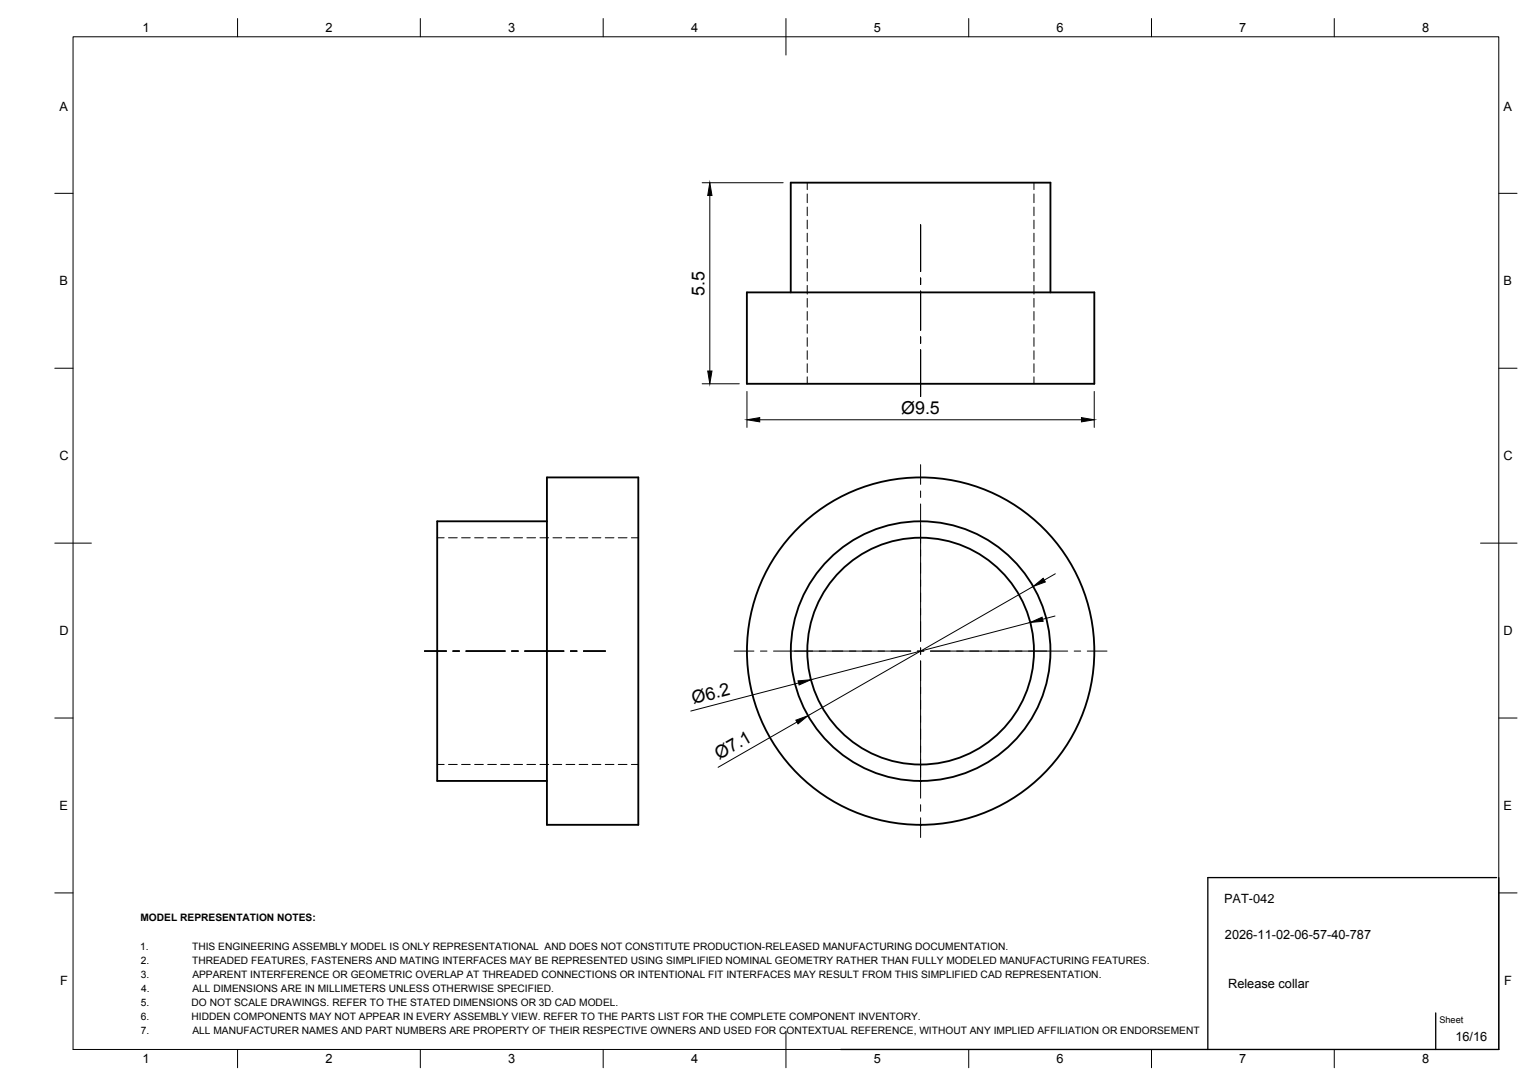
ISO-10303-21;
HEADER;
/* Generated by software containing ST-Developer
 * from STEP Tools, Inc. (www.steptools.com) 
 */

FILE_DESCRIPTION(
/* description */ ('Manifold and mounting hardware'),
/* implementation_level */ '2;1');

FILE_NAME(
/* name */ 'Release collar.step',
/* time_stamp */ '2026-10-28T21:46:49-07:00',
/* author */ (''),
/* organization */ (''),
/* preprocessor_version */ 'ST-DEVELOPER v20.2',
/* originating_system */ 'Autodesk Translation Framework v15.17.0.0',
/* authorisation */ '');

FILE_SCHEMA (('AUTOMOTIVE_DESIGN { 1 0 10303 214 3 1 1 }'));
ENDSEC;

DATA;
#10=MECHANICAL_DESIGN_GEOMETRIC_PRESENTATION_REPRESENTATION('',(#160),#5638);
#132=SHAPE_REPRESENTATION_RELATIONSHIP('SRR','None',#5712,#146);
#146=ADVANCED_BREP_SHAPE_REPRESENTATION('',(#174),#5634);
#160=STYLED_ITEM('',(#5874),#174);
#174=MANIFOLD_SOLID_BREP('Body1',#3150);
#247=FACE_BOUND('',#746,.T.);
#248=FACE_BOUND('',#749,.T.);
#249=FACE_BOUND('',#752,.T.);
#323=CYLINDRICAL_SURFACE('',#3604,0.475);
#324=CYLINDRICAL_SURFACE('',#3608,0.355);
#325=CYLINDRICAL_SURFACE('',#3612,0.31);
#490=FACE_OUTER_BOUND('',#745,.T.);
#491=FACE_OUTER_BOUND('',#747,.T.);
#492=FACE_OUTER_BOUND('',#748,.T.);
#493=FACE_OUTER_BOUND('',#750,.T.);
#494=FACE_OUTER_BOUND('',#751,.T.);
#495=FACE_OUTER_BOUND('',#753,.T.);
#745=EDGE_LOOP('',(#2740));
#746=EDGE_LOOP('',(#2741));
#747=EDGE_LOOP('',(#2742,#2743,#2744,#2745));
#748=EDGE_LOOP('',(#2746));
#749=EDGE_LOOP('',(#2747));
#750=EDGE_LOOP('',(#2748,#2749,#2750,#2751));
#751=EDGE_LOOP('',(#2752));
#752=EDGE_LOOP('',(#2753));
#753=EDGE_LOOP('',(#2754,#2755,#2756,#2757));
#880=CIRCLE('',#3602,0.475);
#881=CIRCLE('',#3603,0.31);
#882=CIRCLE('',#3605,0.475);
#883=CIRCLE('',#3607,0.355);
#884=CIRCLE('',#3609,0.355);
#885=CIRCLE('',#3611,0.31);
#1122=LINE('',#5473,#1369);
#1123=LINE('',#5480,#1370);
#1124=LINE('',#5485,#1371);
#1369=VECTOR('',#4491,0.475);
#1370=VECTOR('',#4500,0.355);
#1371=VECTOR('',#4507,0.31);
#1622=VERTEX_POINT('',#5466);
#1623=VERTEX_POINT('',#5468);
#1624=VERTEX_POINT('',#5471);
#1625=VERTEX_POINT('',#5475);
#1626=VERTEX_POINT('',#5478);
#1627=VERTEX_POINT('',#5482);
#1999=EDGE_CURVE('',#1622,#1622,#880,.T.);
#2000=EDGE_CURVE('',#1623,#1623,#881,.T.);
#2001=EDGE_CURVE('',#1624,#1624,#882,.T.);
#2002=EDGE_CURVE('',#1624,#1622,#1122,.T.);
#2003=EDGE_CURVE('',#1625,#1625,#883,.T.);
#2004=EDGE_CURVE('',#1626,#1626,#884,.T.);
#2005=EDGE_CURVE('',#1626,#1625,#1123,.T.);
#2006=EDGE_CURVE('',#1627,#1627,#885,.T.);
#2007=EDGE_CURVE('',#1627,#1623,#1124,.T.);
#2740=ORIENTED_EDGE('',*,*,#1999,.F.);
#2741=ORIENTED_EDGE('',*,*,#2000,.T.);
#2742=ORIENTED_EDGE('',*,*,#2001,.F.);
#2743=ORIENTED_EDGE('',*,*,#2002,.T.);
#2744=ORIENTED_EDGE('',*,*,#1999,.T.);
#2745=ORIENTED_EDGE('',*,*,#2002,.F.);
#2746=ORIENTED_EDGE('',*,*,#2001,.T.);
#2747=ORIENTED_EDGE('',*,*,#2003,.F.);
#2748=ORIENTED_EDGE('',*,*,#2004,.F.);
#2749=ORIENTED_EDGE('',*,*,#2005,.T.);
#2750=ORIENTED_EDGE('',*,*,#2003,.T.);
#2751=ORIENTED_EDGE('',*,*,#2005,.F.);
#2752=ORIENTED_EDGE('',*,*,#2004,.T.);
#2753=ORIENTED_EDGE('',*,*,#2006,.F.);
#2754=ORIENTED_EDGE('',*,*,#2006,.T.);
#2755=ORIENTED_EDGE('',*,*,#2007,.T.);
#2756=ORIENTED_EDGE('',*,*,#2000,.F.);
#2757=ORIENTED_EDGE('',*,*,#2007,.F.);
#2939=PLANE('',#3601);
#2940=PLANE('',#3606);
#2941=PLANE('',#3610);
#3114=ADVANCED_FACE('',(#490,#247),#2939,.T.);
#3115=ADVANCED_FACE('',(#491),#323,.T.);
#3116=ADVANCED_FACE('',(#492,#248),#2940,.T.);
#3117=ADVANCED_FACE('',(#493),#324,.T.);
#3118=ADVANCED_FACE('',(#494,#249),#2941,.T.);
#3119=ADVANCED_FACE('',(#495),#325,.F.);
#3150=CLOSED_SHELL('',(#3114,#3115,#3116,#3117,#3118,#3119));
#3600=AXIS2_PLACEMENT_3D('',#5464,#4479,#4480);
#3601=AXIS2_PLACEMENT_3D('',#5465,#4481,#4482);
#3602=AXIS2_PLACEMENT_3D('',#5467,#4483,#4484);
#3603=AXIS2_PLACEMENT_3D('',#5469,#4485,#4486);
#3604=AXIS2_PLACEMENT_3D('',#5470,#4487,#4488);
#3605=AXIS2_PLACEMENT_3D('',#5472,#4489,#4490);
#3606=AXIS2_PLACEMENT_3D('',#5474,#4492,#4493);
#3607=AXIS2_PLACEMENT_3D('',#5476,#4494,#4495);
#3608=AXIS2_PLACEMENT_3D('',#5477,#4496,#4497);
#3609=AXIS2_PLACEMENT_3D('',#5479,#4498,#4499);
#3610=AXIS2_PLACEMENT_3D('',#5481,#4501,#4502);
#3611=AXIS2_PLACEMENT_3D('',#5483,#4503,#4504);
#3612=AXIS2_PLACEMENT_3D('',#5484,#4505,#4506);
#4479=DIRECTION('axis',(0.,0.,1.));
#4480=DIRECTION('refdir',(1.,0.,0.));
#4481=DIRECTION('center_axis',(0.,1.,0.));
#4482=DIRECTION('ref_axis',(0.,0.,1.));
#4483=DIRECTION('center_axis',(0.,-1.,0.));
#4484=DIRECTION('ref_axis',(1.,0.,0.));
#4485=DIRECTION('center_axis',(0.,-1.,0.));
#4486=DIRECTION('ref_axis',(1.,0.,0.));
#4487=DIRECTION('center_axis',(0.,-1.,0.));
#4488=DIRECTION('ref_axis',(1.,0.,0.));
#4489=DIRECTION('center_axis',(0.,-1.,0.));
#4490=DIRECTION('ref_axis',(1.,0.,0.));
#4491=DIRECTION('',(0.,1.,0.));
#4492=DIRECTION('center_axis',(0.,-1.,0.));
#4493=DIRECTION('ref_axis',(0.,0.,-1.));
#4494=DIRECTION('center_axis',(0.,-1.,0.));
#4495=DIRECTION('ref_axis',(1.,0.,0.));
#4496=DIRECTION('center_axis',(0.,-1.,0.));
#4497=DIRECTION('ref_axis',(1.,0.,0.));
#4498=DIRECTION('center_axis',(0.,-1.,0.));
#4499=DIRECTION('ref_axis',(1.,0.,0.));
#4500=DIRECTION('',(0.,1.,0.));
#4501=DIRECTION('center_axis',(0.,-1.,0.));
#4502=DIRECTION('ref_axis',(0.,0.,-1.));
#4503=DIRECTION('center_axis',(0.,-1.,0.));
#4504=DIRECTION('ref_axis',(1.,0.,0.));
#4505=DIRECTION('center_axis',(0.,-1.,0.));
#4506=DIRECTION('ref_axis',(1.,0.,0.));
#4507=DIRECTION('',(0.,1.,0.));
#5464=CARTESIAN_POINT('',(0.,0.,0.));
#5465=CARTESIAN_POINT('Origin',(0.475,1.95,0.));
#5466=CARTESIAN_POINT('',(-0.475,1.95,-5.81707229594993E-17));
#5467=CARTESIAN_POINT('Origin',(0.,1.95,0.));
#5468=CARTESIAN_POINT('',(-0.31,1.95,-3.7964050773568E-17));
#5469=CARTESIAN_POINT('Origin',(0.,1.95,0.));
#5470=CARTESIAN_POINT('Origin',(0.,1.825,0.));
#5471=CARTESIAN_POINT('',(-0.475,1.7,-5.81707229594993E-17));
#5472=CARTESIAN_POINT('Origin',(0.,1.7,0.));
#5473=CARTESIAN_POINT('',(-0.475,1.825,-5.81707229594993E-17));
#5474=CARTESIAN_POINT('Origin',(0.355,1.7,0.));
#5475=CARTESIAN_POINT('',(-0.355,1.7,-4.3474961369731E-17));
#5476=CARTESIAN_POINT('Origin',(0.,1.7,0.));
#5477=CARTESIAN_POINT('Origin',(0.,1.55,0.));
#5478=CARTESIAN_POINT('',(-0.355,1.4,-4.3474961369731E-17));
#5479=CARTESIAN_POINT('Origin',(0.,1.4,0.));
#5480=CARTESIAN_POINT('',(-0.355,1.55,-4.3474961369731E-17));
#5481=CARTESIAN_POINT('Origin',(0.31,1.4,0.));
#5482=CARTESIAN_POINT('',(-0.31,1.4,-3.7964050773568E-17));
#5483=CARTESIAN_POINT('Origin',(0.,1.4,0.));
#5484=CARTESIAN_POINT('Origin',(0.,1.675,0.));
#5485=CARTESIAN_POINT('',(-0.31,1.675,-3.7964050773568E-17));
#5617=UNCERTAINTY_MEASURE_WITH_UNIT(LENGTH_MEASURE(0.001),#5639,
'DISTANCE_ACCURACY_VALUE',
'Maximum model space distance between geometric entities at asserted c
onnectivities');
#5621=UNCERTAINTY_MEASURE_WITH_UNIT(LENGTH_MEASURE(0.001),#5639,
'DISTANCE_ACCURACY_VALUE',
'Maximum model space distance between geometric entities at asserted c
onnectivities');
#5634=(
GEOMETRIC_REPRESENTATION_CONTEXT(3)
GLOBAL_UNCERTAINTY_ASSIGNED_CONTEXT((#5617))
GLOBAL_UNIT_ASSIGNED_CONTEXT((#5639,#5641,#5642))
REPRESENTATION_CONTEXT('','3D')
);
#5638=(
GEOMETRIC_REPRESENTATION_CONTEXT(3)
GLOBAL_UNCERTAINTY_ASSIGNED_CONTEXT((#5621))
GLOBAL_UNIT_ASSIGNED_CONTEXT((#5639,#5641,#5642))
REPRESENTATION_CONTEXT('','3D')
);
#5639=(
LENGTH_UNIT()
NAMED_UNIT(*)
SI_UNIT(.CENTI.,.METRE.)
);
#5641=(
NAMED_UNIT(*)
PLANE_ANGLE_UNIT()
SI_UNIT($,.RADIAN.)
);
#5642=(
NAMED_UNIT(*)
SI_UNIT($,.STERADIAN.)
SOLID_ANGLE_UNIT()
);
#5655=SHAPE_DEFINITION_REPRESENTATION(#5671,#5712);
#5671=PRODUCT_DEFINITION_SHAPE('',$,#5729);
#5712=SHAPE_REPRESENTATION('',(#3600),#5634);
#5716=PRODUCT_DEFINITION_CONTEXT('part definition',#5766,'design');
#5729=PRODUCT_DEFINITION('Release collar','Release collar',#5745,
#5716);
#5745=PRODUCT_DEFINITION_FORMATION('',$,#5780);
#5766=APPLICATION_CONTEXT(
'Core Data for Automotive Mechanical Design Process');
#5767=PRODUCT_CONTEXT('part definition',#5766,'mechanical');
#5780=PRODUCT('Release collar','Release collar',
'Release collar',(#5767));
#5868=COLOUR_RGB('Off White',0.89,0.88,0.83);
#5869=FILL_AREA_STYLE_COLOUR('',#5868);
#5870=FILL_AREA_STYLE('',(#5869));
#5871=SURFACE_STYLE_FILL_AREA(#5870);
#5872=SURFACE_SIDE_STYLE('',(#5871));
#5873=SURFACE_STYLE_USAGE(.BOTH.,#5872);
#5874=PRESENTATION_STYLE_ASSIGNMENT((#5873));
ENDSEC;
END-ISO-10303-21;
